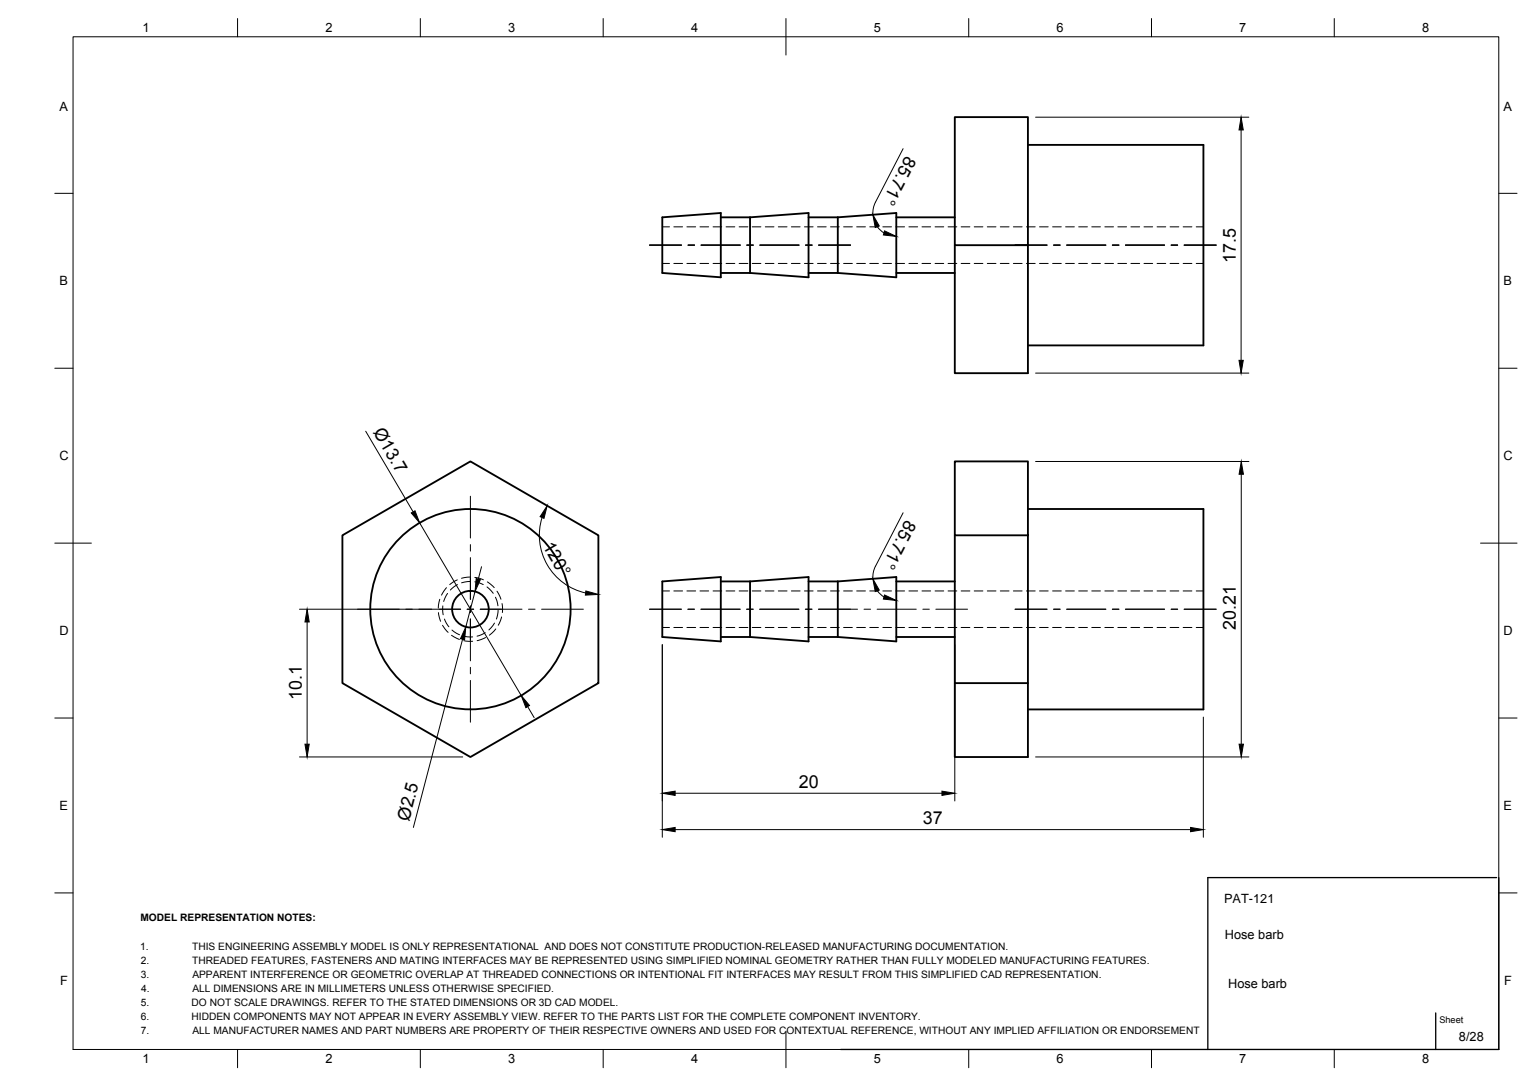
ISO-10303-21;
HEADER;
/* Generated by software containing ST-Developer
 * from STEP Tools, Inc. (www.steptools.com) 
 */

FILE_DESCRIPTION(
/* description */ ('Wall-mounted air drop station'),
/* implementation_level */ '2;1');

FILE_NAME(
/* name */ 'Hose barb.step',
/* time_stamp */ '2026-10-28T22:16:19-07:00',
/* author */ (''),
/* organization */ (''),
/* preprocessor_version */ 'ST-DEVELOPER v20.2',
/* originating_system */ 'Autodesk Translation Framework v15.17.0.0',
/* authorisation */ '');

FILE_SCHEMA (('AUTOMOTIVE_DESIGN { 1 0 10303 214 3 1 1 }'));
ENDSEC;

DATA;
#10=MECHANICAL_DESIGN_GEOMETRIC_PRESENTATION_REPRESENTATION('',(#348),#10517);
#264=CONICAL_SURFACE('',#6349,0.205,0.0748598477107669);
#265=CONICAL_SURFACE('',#6355,0.205,0.0748598477107669);
#266=CONICAL_SURFACE('',#6361,0.205,0.0748598477107669);
#290=SHAPE_REPRESENTATION_RELATIONSHIP('SRR','None',#10647,#319);
#319=ADVANCED_BREP_SHAPE_REPRESENTATION('',(#377),#10491);
#348=STYLED_ITEM('',(#10860),#377);
#377=MANIFOLD_SOLID_BREP('Body1',#5887);
#428=FACE_BOUND('',#1202,.T.);
#429=FACE_BOUND('',#1205,.T.);
#430=FACE_BOUND('',#1209,.T.);
#431=FACE_BOUND('',#1213,.T.);
#432=FACE_BOUND('',#1217,.T.);
#433=FACE_BOUND('',#1225,.T.);
#434=FACE_BOUND('',#1228,.T.);
#567=PLANE('',#6346);
#568=PLANE('',#6351);
#569=PLANE('',#6357);
#570=PLANE('',#6363);
#571=PLANE('',#6369);
#572=PLANE('',#6371);
#573=PLANE('',#6372);
#574=PLANE('',#6373);
#575=PLANE('',#6374);
#576=PLANE('',#6375);
#577=PLANE('',#6376);
#578=PLANE('',#6377);
#579=PLANE('',#6380);
#817=FACE_OUTER_BOUND('',#1201,.T.);
#818=FACE_OUTER_BOUND('',#1203,.T.);
#819=FACE_OUTER_BOUND('',#1204,.T.);
#820=FACE_OUTER_BOUND('',#1206,.T.);
#821=FACE_OUTER_BOUND('',#1207,.T.);
#822=FACE_OUTER_BOUND('',#1208,.T.);
#823=FACE_OUTER_BOUND('',#1210,.T.);
#824=FACE_OUTER_BOUND('',#1211,.T.);
#825=FACE_OUTER_BOUND('',#1212,.T.);
#826=FACE_OUTER_BOUND('',#1214,.T.);
#827=FACE_OUTER_BOUND('',#1215,.T.);
#828=FACE_OUTER_BOUND('',#1216,.T.);
#829=FACE_OUTER_BOUND('',#1218,.T.);
#830=FACE_OUTER_BOUND('',#1219,.T.);
#831=FACE_OUTER_BOUND('',#1220,.T.);
#832=FACE_OUTER_BOUND('',#1221,.T.);
#833=FACE_OUTER_BOUND('',#1222,.T.);
#834=FACE_OUTER_BOUND('',#1223,.T.);
#835=FACE_OUTER_BOUND('',#1224,.T.);
#836=FACE_OUTER_BOUND('',#1226,.T.);
#837=FACE_OUTER_BOUND('',#1227,.T.);
#1201=EDGE_LOOP('',(#4243));
#1202=EDGE_LOOP('',(#4244));
#1203=EDGE_LOOP('',(#4245,#4246,#4247,#4248));
#1204=EDGE_LOOP('',(#4249));
#1205=EDGE_LOOP('',(#4250));
#1206=EDGE_LOOP('',(#4251,#4252,#4253,#4254));
#1207=EDGE_LOOP('',(#4255,#4256,#4257,#4258));
#1208=EDGE_LOOP('',(#4259));
#1209=EDGE_LOOP('',(#4260));
#1210=EDGE_LOOP('',(#4261,#4262,#4263,#4264));
#1211=EDGE_LOOP('',(#4265,#4266,#4267,#4268));
#1212=EDGE_LOOP('',(#4269));
#1213=EDGE_LOOP('',(#4270));
#1214=EDGE_LOOP('',(#4271,#4272,#4273,#4274));
#1215=EDGE_LOOP('',(#4275,#4276,#4277,#4278));
#1216=EDGE_LOOP('',(#4279,#4280,#4281,#4282,#4283,#4284));
#1217=EDGE_LOOP('',(#4285));
#1218=EDGE_LOOP('',(#4286,#4287,#4288,#4289));
#1219=EDGE_LOOP('',(#4290,#4291,#4292,#4293));
#1220=EDGE_LOOP('',(#4294,#4295,#4296,#4297));
#1221=EDGE_LOOP('',(#4298,#4299,#4300,#4301));
#1222=EDGE_LOOP('',(#4302,#4303,#4304,#4305));
#1223=EDGE_LOOP('',(#4306,#4307,#4308,#4309));
#1224=EDGE_LOOP('',(#4310,#4311,#4312,#4313,#4314,#4315));
#1225=EDGE_LOOP('',(#4316));
#1226=EDGE_LOOP('',(#4317,#4318,#4319,#4320));
#1227=EDGE_LOOP('',(#4321));
#1228=EDGE_LOOP('',(#4322));
#1685=LINE('',#9068,#2149);
#1686=LINE('',#9075,#2150);
#1687=LINE('',#9079,#2151);
#1688=LINE('',#9086,#2152);
#1689=LINE('',#9090,#2153);
#1690=LINE('',#9097,#2154);
#1691=LINE('',#9101,#2155);
#1692=LINE('',#9105,#2156);
#1693=LINE('',#9107,#2157);
#1694=LINE('',#9109,#2158);
#1695=LINE('',#9111,#2159);
#1696=LINE('',#9113,#2160);
#1697=LINE('',#9114,#2161);
#1698=LINE('',#9119,#2162);
#1699=LINE('',#9121,#2163);
#1700=LINE('',#9122,#2164);
#1701=LINE('',#9125,#2165);
#1702=LINE('',#9126,#2166);
#1703=LINE('',#9129,#2167);
#1704=LINE('',#9130,#2168);
#1705=LINE('',#9133,#2169);
#1706=LINE('',#9134,#2170);
#1707=LINE('',#9137,#2171);
#1708=LINE('',#9138,#2172);
#1709=LINE('',#9140,#2173);
#1710=LINE('',#9144,#2174);
#2149=VECTOR('',#7249,0.205);
#2150=VECTOR('',#7258,0.19);
#2151=VECTOR('',#7263,0.205);
#2152=VECTOR('',#7272,0.19);
#2153=VECTOR('',#7277,0.205);
#2154=VECTOR('',#7286,0.19);
#2155=VECTOR('',#7291,0.125);
#2156=VECTOR('',#7294,1.);
#2157=VECTOR('',#7295,1.);
#2158=VECTOR('',#7296,1.);
#2159=VECTOR('',#7297,1.);
#2160=VECTOR('',#7298,1.);
#2161=VECTOR('',#7299,1.);
#2162=VECTOR('',#7304,1.);
#2163=VECTOR('',#7305,1.);
#2164=VECTOR('',#7306,1.);
#2165=VECTOR('',#7309,1.);
#2166=VECTOR('',#7310,1.);
#2167=VECTOR('',#7313,1.);
#2168=VECTOR('',#7314,1.);
#2169=VECTOR('',#7317,1.);
#2170=VECTOR('',#7318,1.);
#2171=VECTOR('',#7321,1.);
#2172=VECTOR('',#7322,1.);
#2173=VECTOR('',#7325,1.);
#2174=VECTOR('',#7330,0.685);
#2562=CIRCLE('',#6347,0.19);
#2563=CIRCLE('',#6348,0.125);
#2564=CIRCLE('',#6350,0.22);
#2565=CIRCLE('',#6352,0.19);
#2566=CIRCLE('',#6354,0.19);
#2567=CIRCLE('',#6356,0.22);
#2568=CIRCLE('',#6358,0.19);
#2569=CIRCLE('',#6360,0.19);
#2570=CIRCLE('',#6362,0.22);
#2571=CIRCLE('',#6364,0.19);
#2572=CIRCLE('',#6366,0.19);
#2573=CIRCLE('',#6368,0.125);
#2574=CIRCLE('',#6370,0.685);
#2575=CIRCLE('',#6379,0.685);
#2855=VERTEX_POINT('',#9061);
#2856=VERTEX_POINT('',#9063);
#2857=VERTEX_POINT('',#9066);
#2858=VERTEX_POINT('',#9070);
#2859=VERTEX_POINT('',#9073);
#2860=VERTEX_POINT('',#9077);
#2861=VERTEX_POINT('',#9081);
#2862=VERTEX_POINT('',#9084);
#2863=VERTEX_POINT('',#9088);
#2864=VERTEX_POINT('',#9092);
#2865=VERTEX_POINT('',#9095);
#2866=VERTEX_POINT('',#9099);
#2867=VERTEX_POINT('',#9103);
#2868=VERTEX_POINT('',#9104);
#2869=VERTEX_POINT('',#9106);
#2870=VERTEX_POINT('',#9108);
#2871=VERTEX_POINT('',#9110);
#2872=VERTEX_POINT('',#9112);
#2873=VERTEX_POINT('',#9115);
#2874=VERTEX_POINT('',#9118);
#2875=VERTEX_POINT('',#9120);
#2876=VERTEX_POINT('',#9124);
#2877=VERTEX_POINT('',#9128);
#2878=VERTEX_POINT('',#9132);
#2879=VERTEX_POINT('',#9136);
#2880=VERTEX_POINT('',#9143);
#3379=EDGE_CURVE('',#2855,#2855,#2562,.T.);
#3380=EDGE_CURVE('',#2856,#2856,#2563,.T.);
#3381=EDGE_CURVE('',#2857,#2857,#2564,.T.);
#3382=EDGE_CURVE('',#2857,#2855,#1685,.T.);
#3383=EDGE_CURVE('',#2858,#2858,#2565,.T.);
#3384=EDGE_CURVE('',#2859,#2859,#2566,.T.);
#3385=EDGE_CURVE('',#2859,#2858,#1686,.T.);
#3386=EDGE_CURVE('',#2860,#2860,#2567,.T.);
#3387=EDGE_CURVE('',#2860,#2859,#1687,.T.);
#3388=EDGE_CURVE('',#2861,#2861,#2568,.T.);
#3389=EDGE_CURVE('',#2862,#2862,#2569,.T.);
#3390=EDGE_CURVE('',#2862,#2861,#1688,.T.);
#3391=EDGE_CURVE('',#2863,#2863,#2570,.T.);
#3392=EDGE_CURVE('',#2863,#2862,#1689,.T.);
#3393=EDGE_CURVE('',#2864,#2864,#2571,.T.);
#3394=EDGE_CURVE('',#2865,#2865,#2572,.T.);
#3395=EDGE_CURVE('',#2865,#2864,#1690,.T.);
#3396=EDGE_CURVE('',#2866,#2866,#2573,.T.);
#3397=EDGE_CURVE('',#2866,#2856,#1691,.T.);
#3398=EDGE_CURVE('',#2867,#2868,#1692,.T.);
#3399=EDGE_CURVE('',#2868,#2869,#1693,.T.);
#3400=EDGE_CURVE('',#2869,#2870,#1694,.T.);
#3401=EDGE_CURVE('',#2870,#2871,#1695,.T.);
#3402=EDGE_CURVE('',#2871,#2872,#1696,.T.);
#3403=EDGE_CURVE('',#2872,#2867,#1697,.T.);
#3404=EDGE_CURVE('',#2873,#2873,#2574,.T.);
#3405=EDGE_CURVE('',#2868,#2874,#1698,.T.);
#3406=EDGE_CURVE('',#2875,#2874,#1699,.T.);
#3407=EDGE_CURVE('',#2869,#2875,#1700,.T.);
#3408=EDGE_CURVE('',#2876,#2875,#1701,.T.);
#3409=EDGE_CURVE('',#2870,#2876,#1702,.T.);
#3410=EDGE_CURVE('',#2877,#2876,#1703,.T.);
#3411=EDGE_CURVE('',#2871,#2877,#1704,.T.);
#3412=EDGE_CURVE('',#2878,#2877,#1705,.T.);
#3413=EDGE_CURVE('',#2872,#2878,#1706,.T.);
#3414=EDGE_CURVE('',#2879,#2878,#1707,.T.);
#3415=EDGE_CURVE('',#2867,#2879,#1708,.T.);
#3416=EDGE_CURVE('',#2874,#2879,#1709,.T.);
#3417=EDGE_CURVE('',#2873,#2880,#1710,.T.);
#3418=EDGE_CURVE('',#2880,#2880,#2575,.T.);
#4243=ORIENTED_EDGE('',*,*,#3379,.F.);
#4244=ORIENTED_EDGE('',*,*,#3380,.T.);
#4245=ORIENTED_EDGE('',*,*,#3381,.F.);
#4246=ORIENTED_EDGE('',*,*,#3382,.T.);
#4247=ORIENTED_EDGE('',*,*,#3379,.T.);
#4248=ORIENTED_EDGE('',*,*,#3382,.F.);
#4249=ORIENTED_EDGE('',*,*,#3381,.T.);
#4250=ORIENTED_EDGE('',*,*,#3383,.F.);
#4251=ORIENTED_EDGE('',*,*,#3384,.F.);
#4252=ORIENTED_EDGE('',*,*,#3385,.T.);
#4253=ORIENTED_EDGE('',*,*,#3383,.T.);
#4254=ORIENTED_EDGE('',*,*,#3385,.F.);
#4255=ORIENTED_EDGE('',*,*,#3386,.F.);
#4256=ORIENTED_EDGE('',*,*,#3387,.T.);
#4257=ORIENTED_EDGE('',*,*,#3384,.T.);
#4258=ORIENTED_EDGE('',*,*,#3387,.F.);
#4259=ORIENTED_EDGE('',*,*,#3386,.T.);
#4260=ORIENTED_EDGE('',*,*,#3388,.F.);
#4261=ORIENTED_EDGE('',*,*,#3389,.F.);
#4262=ORIENTED_EDGE('',*,*,#3390,.T.);
#4263=ORIENTED_EDGE('',*,*,#3388,.T.);
#4264=ORIENTED_EDGE('',*,*,#3390,.F.);
#4265=ORIENTED_EDGE('',*,*,#3391,.F.);
#4266=ORIENTED_EDGE('',*,*,#3392,.T.);
#4267=ORIENTED_EDGE('',*,*,#3389,.T.);
#4268=ORIENTED_EDGE('',*,*,#3392,.F.);
#4269=ORIENTED_EDGE('',*,*,#3391,.T.);
#4270=ORIENTED_EDGE('',*,*,#3393,.F.);
#4271=ORIENTED_EDGE('',*,*,#3394,.F.);
#4272=ORIENTED_EDGE('',*,*,#3395,.T.);
#4273=ORIENTED_EDGE('',*,*,#3393,.T.);
#4274=ORIENTED_EDGE('',*,*,#3395,.F.);
#4275=ORIENTED_EDGE('',*,*,#3396,.T.);
#4276=ORIENTED_EDGE('',*,*,#3397,.T.);
#4277=ORIENTED_EDGE('',*,*,#3380,.F.);
#4278=ORIENTED_EDGE('',*,*,#3397,.F.);
#4279=ORIENTED_EDGE('',*,*,#3398,.T.);
#4280=ORIENTED_EDGE('',*,*,#3399,.T.);
#4281=ORIENTED_EDGE('',*,*,#3400,.T.);
#4282=ORIENTED_EDGE('',*,*,#3401,.T.);
#4283=ORIENTED_EDGE('',*,*,#3402,.T.);
#4284=ORIENTED_EDGE('',*,*,#3403,.T.);
#4285=ORIENTED_EDGE('',*,*,#3404,.T.);
#4286=ORIENTED_EDGE('',*,*,#3399,.F.);
#4287=ORIENTED_EDGE('',*,*,#3405,.T.);
#4288=ORIENTED_EDGE('',*,*,#3406,.F.);
#4289=ORIENTED_EDGE('',*,*,#3407,.F.);
#4290=ORIENTED_EDGE('',*,*,#3400,.F.);
#4291=ORIENTED_EDGE('',*,*,#3407,.T.);
#4292=ORIENTED_EDGE('',*,*,#3408,.F.);
#4293=ORIENTED_EDGE('',*,*,#3409,.F.);
#4294=ORIENTED_EDGE('',*,*,#3401,.F.);
#4295=ORIENTED_EDGE('',*,*,#3409,.T.);
#4296=ORIENTED_EDGE('',*,*,#3410,.F.);
#4297=ORIENTED_EDGE('',*,*,#3411,.F.);
#4298=ORIENTED_EDGE('',*,*,#3402,.F.);
#4299=ORIENTED_EDGE('',*,*,#3411,.T.);
#4300=ORIENTED_EDGE('',*,*,#3412,.F.);
#4301=ORIENTED_EDGE('',*,*,#3413,.F.);
#4302=ORIENTED_EDGE('',*,*,#3403,.F.);
#4303=ORIENTED_EDGE('',*,*,#3413,.T.);
#4304=ORIENTED_EDGE('',*,*,#3414,.F.);
#4305=ORIENTED_EDGE('',*,*,#3415,.F.);
#4306=ORIENTED_EDGE('',*,*,#3398,.F.);
#4307=ORIENTED_EDGE('',*,*,#3415,.T.);
#4308=ORIENTED_EDGE('',*,*,#3416,.F.);
#4309=ORIENTED_EDGE('',*,*,#3405,.F.);
#4310=ORIENTED_EDGE('',*,*,#3416,.T.);
#4311=ORIENTED_EDGE('',*,*,#3414,.T.);
#4312=ORIENTED_EDGE('',*,*,#3412,.T.);
#4313=ORIENTED_EDGE('',*,*,#3410,.T.);
#4314=ORIENTED_EDGE('',*,*,#3408,.T.);
#4315=ORIENTED_EDGE('',*,*,#3406,.T.);
#4316=ORIENTED_EDGE('',*,*,#3394,.T.);
#4317=ORIENTED_EDGE('',*,*,#3404,.F.);
#4318=ORIENTED_EDGE('',*,*,#3417,.T.);
#4319=ORIENTED_EDGE('',*,*,#3418,.T.);
#4320=ORIENTED_EDGE('',*,*,#3417,.F.);
#4321=ORIENTED_EDGE('',*,*,#3418,.F.);
#4322=ORIENTED_EDGE('',*,*,#3396,.F.);
#5452=CYLINDRICAL_SURFACE('',#6353,0.19);
#5453=CYLINDRICAL_SURFACE('',#6359,0.19);
#5454=CYLINDRICAL_SURFACE('',#6365,0.19);
#5455=CYLINDRICAL_SURFACE('',#6367,0.125);
#5456=CYLINDRICAL_SURFACE('',#6378,0.685);
#5590=ADVANCED_FACE('',(#817,#428),#567,.T.);
#5591=ADVANCED_FACE('',(#818),#264,.T.);
#5592=ADVANCED_FACE('',(#819,#429),#568,.T.);
#5593=ADVANCED_FACE('',(#820),#5452,.T.);
#5594=ADVANCED_FACE('',(#821),#265,.T.);
#5595=ADVANCED_FACE('',(#822,#430),#569,.T.);
#5596=ADVANCED_FACE('',(#823),#5453,.T.);
#5597=ADVANCED_FACE('',(#824),#266,.T.);
#5598=ADVANCED_FACE('',(#825,#431),#570,.T.);
#5599=ADVANCED_FACE('',(#826),#5454,.T.);
#5600=ADVANCED_FACE('',(#827),#5455,.F.);
#5601=ADVANCED_FACE('',(#828,#432),#571,.F.);
#5602=ADVANCED_FACE('',(#829),#572,.T.);
#5603=ADVANCED_FACE('',(#830),#573,.T.);
#5604=ADVANCED_FACE('',(#831),#574,.T.);
#5605=ADVANCED_FACE('',(#832),#575,.T.);
#5606=ADVANCED_FACE('',(#833),#576,.T.);
#5607=ADVANCED_FACE('',(#834),#577,.T.);
#5608=ADVANCED_FACE('',(#835,#433),#578,.T.);
#5609=ADVANCED_FACE('',(#836),#5456,.T.);
#5610=ADVANCED_FACE('',(#837,#434),#579,.F.);
#5887=CLOSED_SHELL('',(#5590,#5591,#5592,#5593,#5594,#5595,#5596,#5597,
#5598,#5599,#5600,#5601,#5602,#5603,#5604,#5605,#5606,#5607,#5608,#5609,
#5610));
#6345=AXIS2_PLACEMENT_3D('',#9059,#7237,#7238);
#6346=AXIS2_PLACEMENT_3D('',#9060,#7239,#7240);
#6347=AXIS2_PLACEMENT_3D('',#9062,#7241,#7242);
#6348=AXIS2_PLACEMENT_3D('',#9064,#7243,#7244);
#6349=AXIS2_PLACEMENT_3D('',#9065,#7245,#7246);
#6350=AXIS2_PLACEMENT_3D('',#9067,#7247,#7248);
#6351=AXIS2_PLACEMENT_3D('',#9069,#7250,#7251);
#6352=AXIS2_PLACEMENT_3D('',#9071,#7252,#7253);
#6353=AXIS2_PLACEMENT_3D('',#9072,#7254,#7255);
#6354=AXIS2_PLACEMENT_3D('',#9074,#7256,#7257);
#6355=AXIS2_PLACEMENT_3D('',#9076,#7259,#7260);
#6356=AXIS2_PLACEMENT_3D('',#9078,#7261,#7262);
#6357=AXIS2_PLACEMENT_3D('',#9080,#7264,#7265);
#6358=AXIS2_PLACEMENT_3D('',#9082,#7266,#7267);
#6359=AXIS2_PLACEMENT_3D('',#9083,#7268,#7269);
#6360=AXIS2_PLACEMENT_3D('',#9085,#7270,#7271);
#6361=AXIS2_PLACEMENT_3D('',#9087,#7273,#7274);
#6362=AXIS2_PLACEMENT_3D('',#9089,#7275,#7276);
#6363=AXIS2_PLACEMENT_3D('',#9091,#7278,#7279);
#6364=AXIS2_PLACEMENT_3D('',#9093,#7280,#7281);
#6365=AXIS2_PLACEMENT_3D('',#9094,#7282,#7283);
#6366=AXIS2_PLACEMENT_3D('',#9096,#7284,#7285);
#6367=AXIS2_PLACEMENT_3D('',#9098,#7287,#7288);
#6368=AXIS2_PLACEMENT_3D('',#9100,#7289,#7290);
#6369=AXIS2_PLACEMENT_3D('',#9102,#7292,#7293);
#6370=AXIS2_PLACEMENT_3D('',#9116,#7300,#7301);
#6371=AXIS2_PLACEMENT_3D('',#9117,#7302,#7303);
#6372=AXIS2_PLACEMENT_3D('',#9123,#7307,#7308);
#6373=AXIS2_PLACEMENT_3D('',#9127,#7311,#7312);
#6374=AXIS2_PLACEMENT_3D('',#9131,#7315,#7316);
#6375=AXIS2_PLACEMENT_3D('',#9135,#7319,#7320);
#6376=AXIS2_PLACEMENT_3D('',#9139,#7323,#7324);
#6377=AXIS2_PLACEMENT_3D('',#9141,#7326,#7327);
#6378=AXIS2_PLACEMENT_3D('',#9142,#7328,#7329);
#6379=AXIS2_PLACEMENT_3D('',#9145,#7331,#7332);
#6380=AXIS2_PLACEMENT_3D('',#9146,#7333,#7334);
#7237=DIRECTION('axis',(0.,0.,1.));
#7238=DIRECTION('refdir',(1.,0.,0.));
#7239=DIRECTION('center_axis',(0.,1.,0.));
#7240=DIRECTION('ref_axis',(0.,0.,1.));
#7241=DIRECTION('center_axis',(0.,-1.,0.));
#7242=DIRECTION('ref_axis',(1.,0.,0.));
#7243=DIRECTION('center_axis',(0.,-1.,0.));
#7244=DIRECTION('ref_axis',(1.,0.,0.));
#7245=DIRECTION('center_axis',(0.,-1.,0.));
#7246=DIRECTION('ref_axis',(1.,0.,0.));
#7247=DIRECTION('center_axis',(0.,-1.,0.));
#7248=DIRECTION('ref_axis',(1.,0.,0.));
#7249=DIRECTION('',(0.0747899482416342,0.997199309888456,9.15912707225136E-18));
#7250=DIRECTION('center_axis',(0.,-1.,0.));
#7251=DIRECTION('ref_axis',(0.,0.,-1.));
#7252=DIRECTION('center_axis',(0.,-1.,0.));
#7253=DIRECTION('ref_axis',(1.,0.,0.));
#7254=DIRECTION('center_axis',(0.,-1.,0.));
#7255=DIRECTION('ref_axis',(1.,0.,0.));
#7256=DIRECTION('center_axis',(0.,-1.,0.));
#7257=DIRECTION('ref_axis',(1.,0.,0.));
#7258=DIRECTION('',(0.,1.,0.));
#7259=DIRECTION('center_axis',(0.,-1.,0.));
#7260=DIRECTION('ref_axis',(1.,0.,0.));
#7261=DIRECTION('center_axis',(0.,-1.,0.));
#7262=DIRECTION('ref_axis',(1.,0.,0.));
#7263=DIRECTION('',(0.0747899482416342,0.997199309888456,9.15912707225136E-18));
#7264=DIRECTION('center_axis',(0.,-1.,0.));
#7265=DIRECTION('ref_axis',(0.,0.,-1.));
#7266=DIRECTION('center_axis',(0.,-1.,0.));
#7267=DIRECTION('ref_axis',(1.,0.,0.));
#7268=DIRECTION('center_axis',(0.,-1.,0.));
#7269=DIRECTION('ref_axis',(1.,0.,0.));
#7270=DIRECTION('center_axis',(0.,-1.,0.));
#7271=DIRECTION('ref_axis',(1.,0.,0.));
#7272=DIRECTION('',(0.,1.,0.));
#7273=DIRECTION('center_axis',(0.,-1.,0.));
#7274=DIRECTION('ref_axis',(1.,0.,0.));
#7275=DIRECTION('center_axis',(0.,-1.,0.));
#7276=DIRECTION('ref_axis',(1.,0.,0.));
#7277=DIRECTION('',(0.0747899482416342,0.997199309888456,9.15912707225136E-18));
#7278=DIRECTION('center_axis',(0.,-1.,0.));
#7279=DIRECTION('ref_axis',(0.,0.,-1.));
#7280=DIRECTION('center_axis',(0.,-1.,0.));
#7281=DIRECTION('ref_axis',(1.,0.,0.));
#7282=DIRECTION('center_axis',(0.,-1.,0.));
#7283=DIRECTION('ref_axis',(1.,0.,0.));
#7284=DIRECTION('center_axis',(0.,-1.,0.));
#7285=DIRECTION('ref_axis',(1.,0.,0.));
#7286=DIRECTION('',(0.,1.,0.));
#7287=DIRECTION('center_axis',(0.,-1.,0.));
#7288=DIRECTION('ref_axis',(1.,0.,0.));
#7289=DIRECTION('center_axis',(0.,-1.,0.));
#7290=DIRECTION('ref_axis',(1.,0.,0.));
#7291=DIRECTION('',(0.,1.,0.));
#7292=DIRECTION('center_axis',(0.,1.,0.));
#7293=DIRECTION('ref_axis',(1.,0.,0.));
#7294=DIRECTION('',(1.,0.,0.));
#7295=DIRECTION('',(0.5,0.,0.866025403784439));
#7296=DIRECTION('',(-0.5,0.,0.866025403784439));
#7297=DIRECTION('',(-1.,0.,0.));
#7298=DIRECTION('',(-0.5,0.,-0.866025403784439));
#7299=DIRECTION('',(0.5,0.,-0.866025403784439));
#7300=DIRECTION('center_axis',(0.,1.,0.));
#7301=DIRECTION('ref_axis',(1.,0.,0.));
#7302=DIRECTION('center_axis',(0.866025403784439,0.,-0.5));
#7303=DIRECTION('ref_axis',(-0.5,0.,-0.866025403784439));
#7304=DIRECTION('',(0.,1.,0.));
#7305=DIRECTION('',(-0.5,0.,-0.866025403784439));
#7306=DIRECTION('',(0.,1.,0.));
#7307=DIRECTION('center_axis',(0.866025403784439,0.,0.5));
#7308=DIRECTION('ref_axis',(0.5,0.,-0.866025403784439));
#7309=DIRECTION('',(0.5,0.,-0.866025403784439));
#7310=DIRECTION('',(0.,1.,0.));
#7311=DIRECTION('center_axis',(0.,0.,1.));
#7312=DIRECTION('ref_axis',(1.,0.,0.));
#7313=DIRECTION('',(1.,0.,0.));
#7314=DIRECTION('',(0.,1.,0.));
#7315=DIRECTION('center_axis',(-0.866025403784439,0.,0.5));
#7316=DIRECTION('ref_axis',(0.5,0.,0.866025403784439));
#7317=DIRECTION('',(0.5,0.,0.866025403784439));
#7318=DIRECTION('',(0.,1.,0.));
#7319=DIRECTION('center_axis',(-0.866025403784439,0.,-0.5));
#7320=DIRECTION('ref_axis',(-0.5,0.,0.866025403784439));
#7321=DIRECTION('',(-0.5,0.,0.866025403784439));
#7322=DIRECTION('',(0.,1.,0.));
#7323=DIRECTION('center_axis',(0.,0.,-1.));
#7324=DIRECTION('ref_axis',(-1.,0.,0.));
#7325=DIRECTION('',(-1.,0.,0.));
#7326=DIRECTION('center_axis',(0.,1.,0.));
#7327=DIRECTION('ref_axis',(0.,0.,1.));
#7328=DIRECTION('center_axis',(0.,1.,0.));
#7329=DIRECTION('ref_axis',(1.,0.,0.));
#7330=DIRECTION('',(0.,-1.,0.));
#7331=DIRECTION('center_axis',(0.,1.,0.));
#7332=DIRECTION('ref_axis',(1.,0.,0.));
#7333=DIRECTION('center_axis',(0.,1.,0.));
#7334=DIRECTION('ref_axis',(1.,0.,0.));
#9059=CARTESIAN_POINT('',(0.,0.,0.));
#9060=CARTESIAN_POINT('Origin',(0.19,11.,5.));
#9061=CARTESIAN_POINT('',(-0.19,11.,5.));
#9062=CARTESIAN_POINT('Origin',(0.,11.,5.));
#9063=CARTESIAN_POINT('',(-0.125,11.,5.));
#9064=CARTESIAN_POINT('Origin',(0.,11.,5.));
#9065=CARTESIAN_POINT('Origin',(0.,10.8,5.));
#9066=CARTESIAN_POINT('',(-0.22,10.6,5.));
#9067=CARTESIAN_POINT('Origin',(0.,10.6,5.));
#9068=CARTESIAN_POINT('',(-0.205,10.8,5.));
#9069=CARTESIAN_POINT('Origin',(0.19,10.6,5.));
#9070=CARTESIAN_POINT('',(-0.19,10.6,5.));
#9071=CARTESIAN_POINT('Origin',(0.,10.6,5.));
#9072=CARTESIAN_POINT('Origin',(0.,10.5,5.));
#9073=CARTESIAN_POINT('',(-0.19,10.4,5.));
#9074=CARTESIAN_POINT('Origin',(0.,10.4,5.));
#9075=CARTESIAN_POINT('',(-0.19,10.5,5.));
#9076=CARTESIAN_POINT('Origin',(0.,10.2,5.));
#9077=CARTESIAN_POINT('',(-0.22,10.,5.));
#9078=CARTESIAN_POINT('Origin',(0.,10.,5.));
#9079=CARTESIAN_POINT('',(-0.205,10.2,5.));
#9080=CARTESIAN_POINT('Origin',(0.19,10.,5.));
#9081=CARTESIAN_POINT('',(-0.19,10.,5.));
#9082=CARTESIAN_POINT('Origin',(0.,10.,5.));
#9083=CARTESIAN_POINT('Origin',(0.,9.9,5.));
#9084=CARTESIAN_POINT('',(-0.19,9.8,5.));
#9085=CARTESIAN_POINT('Origin',(0.,9.8,5.));
#9086=CARTESIAN_POINT('',(-0.19,9.9,5.));
#9087=CARTESIAN_POINT('Origin',(0.,9.6,5.));
#9088=CARTESIAN_POINT('',(-0.22,9.4,5.));
#9089=CARTESIAN_POINT('Origin',(0.,9.4,5.));
#9090=CARTESIAN_POINT('',(-0.205,9.6,5.));
#9091=CARTESIAN_POINT('Origin',(0.19,9.4,5.));
#9092=CARTESIAN_POINT('',(-0.19,9.4,5.));
#9093=CARTESIAN_POINT('Origin',(0.,9.4,5.));
#9094=CARTESIAN_POINT('Origin',(0.,9.2,5.));
#9095=CARTESIAN_POINT('',(-0.19,9.,5.));
#9096=CARTESIAN_POINT('Origin',(0.,9.,5.));
#9097=CARTESIAN_POINT('',(-0.19,9.2,5.));
#9098=CARTESIAN_POINT('Origin',(0.,10.,5.));
#9099=CARTESIAN_POINT('',(-0.125,7.3,5.));
#9100=CARTESIAN_POINT('Origin',(0.,7.3,5.));
#9101=CARTESIAN_POINT('',(-0.125,10.,5.));
#9102=CARTESIAN_POINT('Origin',(0.,8.5,5.));
#9103=CARTESIAN_POINT('',(-0.505181485540923,8.5,4.125));
#9104=CARTESIAN_POINT('',(0.505181485540923,8.5,4.125));
#9105=CARTESIAN_POINT('',(-0.505181485540923,8.5,4.125));
#9106=CARTESIAN_POINT('',(1.01036297108185,8.5,5.));
#9107=CARTESIAN_POINT('',(0.505181485540923,8.5,4.125));
#9108=CARTESIAN_POINT('',(0.505181485540923,8.5,5.875));
#9109=CARTESIAN_POINT('',(1.01036297108185,8.5,5.));
#9110=CARTESIAN_POINT('',(-0.505181485540922,8.5,5.875));
#9111=CARTESIAN_POINT('',(0.505181485540923,8.5,5.875));
#9112=CARTESIAN_POINT('',(-1.01036297108185,8.5,5.));
#9113=CARTESIAN_POINT('',(-0.505181485540922,8.5,5.875));
#9114=CARTESIAN_POINT('',(-1.01036297108185,8.5,5.));
#9115=CARTESIAN_POINT('',(-0.685,8.5,5.));
#9116=CARTESIAN_POINT('Origin',(0.,8.5,5.));
#9117=CARTESIAN_POINT('Origin',(1.01036297108184,8.5,5.));
#9118=CARTESIAN_POINT('',(0.505181485540923,9.,4.125));
#9119=CARTESIAN_POINT('',(0.505181485540923,8.5,4.125));
#9120=CARTESIAN_POINT('',(1.01036297108185,9.,5.));
#9121=CARTESIAN_POINT('',(0.505181485540923,9.,4.125));
#9122=CARTESIAN_POINT('',(1.01036297108185,8.5,5.));
#9123=CARTESIAN_POINT('Origin',(0.505181485540923,8.5,5.875));
#9124=CARTESIAN_POINT('',(0.505181485540923,9.,5.875));
#9125=CARTESIAN_POINT('',(1.01036297108185,9.,5.));
#9126=CARTESIAN_POINT('',(0.505181485540923,8.5,5.875));
#9127=CARTESIAN_POINT('Origin',(-0.505181485540922,8.5,5.875));
#9128=CARTESIAN_POINT('',(-0.505181485540922,9.,5.875));
#9129=CARTESIAN_POINT('',(0.505181485540923,9.,5.875));
#9130=CARTESIAN_POINT('',(-0.505181485540922,8.5,5.875));
#9131=CARTESIAN_POINT('Origin',(-1.01036297108185,8.5,5.));
#9132=CARTESIAN_POINT('',(-1.01036297108185,9.,5.));
#9133=CARTESIAN_POINT('',(-0.505181485540922,9.,5.875));
#9134=CARTESIAN_POINT('',(-1.01036297108185,8.5,5.));
#9135=CARTESIAN_POINT('Origin',(-0.505181485540923,8.5,4.125));
#9136=CARTESIAN_POINT('',(-0.505181485540923,9.,4.125));
#9137=CARTESIAN_POINT('',(-1.01036297108185,9.,5.));
#9138=CARTESIAN_POINT('',(-0.505181485540923,8.5,4.125));
#9139=CARTESIAN_POINT('Origin',(0.505181485540923,8.5,4.125));
#9140=CARTESIAN_POINT('',(-0.505181485540923,9.,4.125));
#9141=CARTESIAN_POINT('Origin',(0.,9.,5.));
#9142=CARTESIAN_POINT('Origin',(0.,7.3,5.));
#9143=CARTESIAN_POINT('',(-0.685,7.3,5.));
#9144=CARTESIAN_POINT('',(-0.685,7.3,5.));
#9145=CARTESIAN_POINT('Origin',(0.,7.3,5.));
#9146=CARTESIAN_POINT('Origin',(0.,7.3,5.));
#10458=UNCERTAINTY_MEASURE_WITH_UNIT(LENGTH_MEASURE(0.001),#10518,
'DISTANCE_ACCURACY_VALUE',
'Maximum model space distance between geometric entities at asserted c
onnectivities');
#10484=UNCERTAINTY_MEASURE_WITH_UNIT(LENGTH_MEASURE(0.001),#10518,
'DISTANCE_ACCURACY_VALUE',
'Maximum model space distance between geometric entities at asserted c
onnectivities');
#10491=(
GEOMETRIC_REPRESENTATION_CONTEXT(3)
GLOBAL_UNCERTAINTY_ASSIGNED_CONTEXT((#10458))
GLOBAL_UNIT_ASSIGNED_CONTEXT((#10518,#10520,#10521))
REPRESENTATION_CONTEXT('','3D')
);
#10517=(
GEOMETRIC_REPRESENTATION_CONTEXT(3)
GLOBAL_UNCERTAINTY_ASSIGNED_CONTEXT((#10484))
GLOBAL_UNIT_ASSIGNED_CONTEXT((#10518,#10520,#10521))
REPRESENTATION_CONTEXT('','3D')
);
#10518=(
LENGTH_UNIT()
NAMED_UNIT(*)
SI_UNIT(.CENTI.,.METRE.)
);
#10520=(
NAMED_UNIT(*)
PLANE_ANGLE_UNIT()
SI_UNIT($,.RADIAN.)
);
#10521=(
NAMED_UNIT(*)
SI_UNIT($,.STERADIAN.)
SOLID_ANGLE_UNIT()
);
#10528=SHAPE_DEFINITION_REPRESENTATION(#10560,#10647);
#10560=PRODUCT_DEFINITION_SHAPE('',$,#10680);
#10647=SHAPE_REPRESENTATION('',(#6345),#10491);
#10673=PRODUCT_DEFINITION_CONTEXT('part definition',#10771,'design');
#10680=PRODUCT_DEFINITION('Hose barb','Hose barb',#10712,#10673);
#10712=PRODUCT_DEFINITION_FORMATION('',$,#10779);
#10771=APPLICATION_CONTEXT(
'Core Data for Automotive Mechanical Design Process');
#10772=PRODUCT_CONTEXT('part definition',#10771,'mechanical');
#10779=PRODUCT('Hose barb','Hose barb','Hose barb',(#10772));
#10854=COLOUR_RGB('Light Blue',0.38,0.62,0.78);
#10855=FILL_AREA_STYLE_COLOUR('',#10854);
#10856=FILL_AREA_STYLE('',(#10855));
#10857=SURFACE_STYLE_FILL_AREA(#10856);
#10858=SURFACE_SIDE_STYLE('',(#10857));
#10859=SURFACE_STYLE_USAGE(.BOTH.,#10858);
#10860=PRESENTATION_STYLE_ASSIGNMENT((#10859));
ENDSEC;
END-ISO-10303-21;
